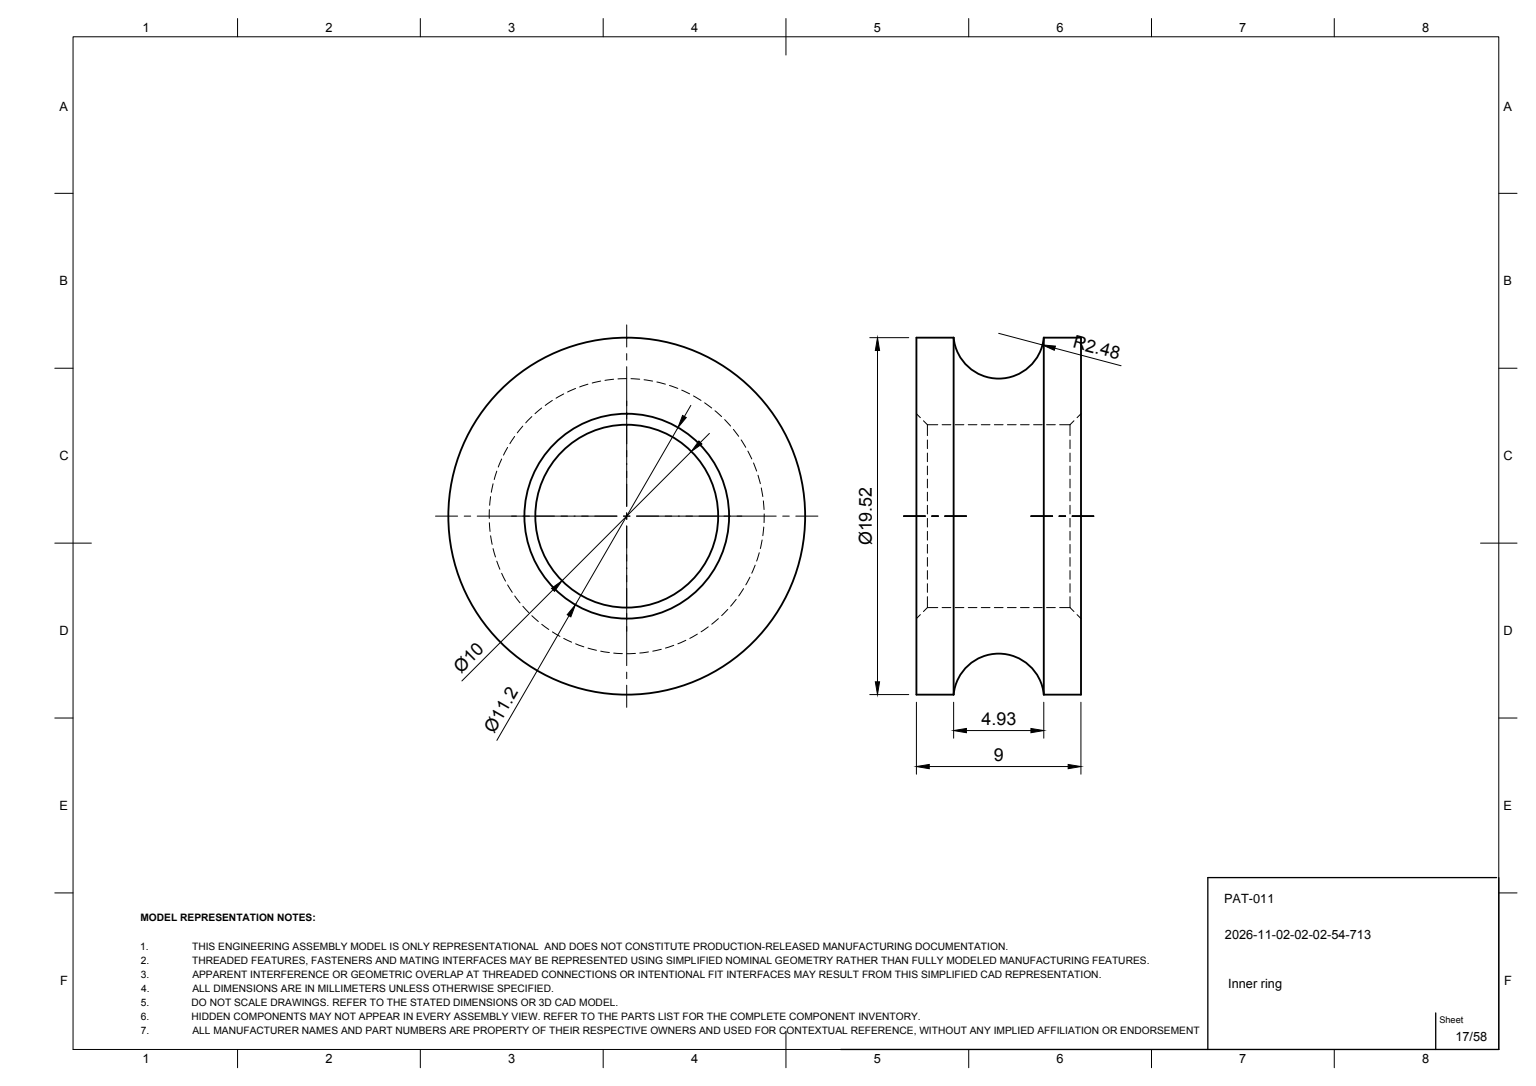
ISO-10303-21;
HEADER;
/* Generated by software containing ST-Developer
 * from STEP Tools, Inc. (www.steptools.com) 
 */

FILE_DESCRIPTION(
/* description */ ('Belt tension measurement rig'),
/* implementation_level */ '2;1');

FILE_NAME(
/* name */ 'Inner ring.step',
/* time_stamp */ '2026-10-28T03:24:44-07:00',
/* author */ (''),
/* organization */ (''),
/* preprocessor_version */ 'ST-DEVELOPER v20.2',
/* originating_system */ 'Autodesk Translation Framework v15.17.0.0',
/* authorisation */ '');

FILE_SCHEMA (('AUTOMOTIVE_DESIGN { 1 0 10303 214 3 1 1 }'));
ENDSEC;

DATA;
#10=MECHANICAL_DESIGN_GEOMETRIC_PRESENTATION_REPRESENTATION('',(#706),#23587);
#467=CONICAL_SURFACE('',#13234,0.53,0.785398163397448);
#468=CONICAL_SURFACE('',#13241,0.53,0.785398163397448);
#487=TOROIDAL_SURFACE('',#13223,1.,0.247676);
#596=SHAPE_REPRESENTATION_RELATIONSHIP('SRR','None',#23842,#651);
#651=ADVANCED_BREP_SHAPE_REPRESENTATION('',(#776),#23540);
#706=STYLED_ITEM('',(#24211),#776);
#776=MANIFOLD_SOLID_BREP('Body1',#12211);
#907=FACE_BOUND('',#2316,.T.);
#908=FACE_BOUND('',#2319,.T.);
#1138=PLANE('',#13236);
#1139=PLANE('',#13239);
#1529=FACE_OUTER_BOUND('',#2311,.T.);
#1530=FACE_OUTER_BOUND('',#2312,.T.);
#1531=FACE_OUTER_BOUND('',#2313,.T.);
#1532=FACE_OUTER_BOUND('',#2314,.T.);
#1533=FACE_OUTER_BOUND('',#2315,.T.);
#1534=FACE_OUTER_BOUND('',#2317,.T.);
#1535=FACE_OUTER_BOUND('',#2318,.T.);
#1536=FACE_OUTER_BOUND('',#2320,.T.);
#2311=EDGE_LOOP('',(#8684,#8685,#8686,#8687,#8688,#8689));
#2312=EDGE_LOOP('',(#8690,#8691,#8692,#8693,#8694));
#2313=EDGE_LOOP('',(#8695,#8696,#8697,#8698));
#2314=EDGE_LOOP('',(#8699,#8700,#8701,#8702));
#2315=EDGE_LOOP('',(#8703));
#2316=EDGE_LOOP('',(#8704));
#2317=EDGE_LOOP('',(#8705,#8706,#8707,#8708,#8709));
#2318=EDGE_LOOP('',(#8710));
#2319=EDGE_LOOP('',(#8711));
#2320=EDGE_LOOP('',(#8712,#8713,#8714,#8715));
#3185=LINE('',#19448,#3936);
#3186=LINE('',#19454,#3937);
#3187=LINE('',#19458,#3938);
#3188=LINE('',#19464,#3939);
#3189=LINE('',#19469,#3940);
#3936=VECTOR('',#15442,0.976185);
#3937=VECTOR('',#15449,0.5);
#3938=VECTOR('',#15454,0.53);
#3939=VECTOR('',#15463,0.976185);
#3940=VECTOR('',#15470,0.53);
#4622=CIRCLE('',#13224,0.976185);
#4623=CIRCLE('',#13225,0.976185);
#4624=CIRCLE('',#13226,0.247676);
#4625=CIRCLE('',#13227,0.976185);
#4626=CIRCLE('',#13228,0.976185);
#4627=CIRCLE('',#13230,0.976185);
#4628=CIRCLE('',#13232,0.5);
#4629=CIRCLE('',#13233,0.5);
#4630=CIRCLE('',#13235,0.56);
#4631=CIRCLE('',#13238,0.976185);
#4632=CIRCLE('',#13240,0.56);
#5484=VERTEX_POINT('',#19437);
#5485=VERTEX_POINT('',#19438);
#5486=VERTEX_POINT('',#19441);
#5487=VERTEX_POINT('',#19443);
#5488=VERTEX_POINT('',#19447);
#5489=VERTEX_POINT('',#19451);
#5490=VERTEX_POINT('',#19453);
#5491=VERTEX_POINT('',#19457);
#5492=VERTEX_POINT('',#19462);
#5493=VERTEX_POINT('',#19466);
#6701=EDGE_CURVE('',#5484,#5485,#4622,.T.);
#6702=EDGE_CURVE('',#5485,#5484,#4623,.T.);
#6703=EDGE_CURVE('',#5485,#5486,#4624,.T.);
#6704=EDGE_CURVE('',#5487,#5486,#4625,.T.);
#6705=EDGE_CURVE('',#5486,#5487,#4626,.T.);
#6706=EDGE_CURVE('',#5487,#5488,#3185,.T.);
#6707=EDGE_CURVE('',#5488,#5488,#4627,.T.);
#6708=EDGE_CURVE('',#5489,#5489,#4628,.T.);
#6709=EDGE_CURVE('',#5489,#5490,#3186,.T.);
#6710=EDGE_CURVE('',#5490,#5490,#4629,.T.);
#6711=EDGE_CURVE('',#5490,#5491,#3187,.T.);
#6712=EDGE_CURVE('',#5491,#5491,#4630,.T.);
#6713=EDGE_CURVE('',#5492,#5492,#4631,.T.);
#6714=EDGE_CURVE('',#5492,#5484,#3188,.T.);
#6715=EDGE_CURVE('',#5493,#5493,#4632,.T.);
#6716=EDGE_CURVE('',#5493,#5489,#3189,.T.);
#8684=ORIENTED_EDGE('',*,*,#6701,.F.);
#8685=ORIENTED_EDGE('',*,*,#6702,.F.);
#8686=ORIENTED_EDGE('',*,*,#6703,.T.);
#8687=ORIENTED_EDGE('',*,*,#6704,.F.);
#8688=ORIENTED_EDGE('',*,*,#6705,.F.);
#8689=ORIENTED_EDGE('',*,*,#6703,.F.);
#8690=ORIENTED_EDGE('',*,*,#6704,.T.);
#8691=ORIENTED_EDGE('',*,*,#6705,.T.);
#8692=ORIENTED_EDGE('',*,*,#6706,.T.);
#8693=ORIENTED_EDGE('',*,*,#6707,.T.);
#8694=ORIENTED_EDGE('',*,*,#6706,.F.);
#8695=ORIENTED_EDGE('',*,*,#6708,.T.);
#8696=ORIENTED_EDGE('',*,*,#6709,.T.);
#8697=ORIENTED_EDGE('',*,*,#6710,.F.);
#8698=ORIENTED_EDGE('',*,*,#6709,.F.);
#8699=ORIENTED_EDGE('',*,*,#6710,.T.);
#8700=ORIENTED_EDGE('',*,*,#6711,.T.);
#8701=ORIENTED_EDGE('',*,*,#6712,.F.);
#8702=ORIENTED_EDGE('',*,*,#6711,.F.);
#8703=ORIENTED_EDGE('',*,*,#6707,.F.);
#8704=ORIENTED_EDGE('',*,*,#6712,.T.);
#8705=ORIENTED_EDGE('',*,*,#6713,.F.);
#8706=ORIENTED_EDGE('',*,*,#6714,.T.);
#8707=ORIENTED_EDGE('',*,*,#6701,.T.);
#8708=ORIENTED_EDGE('',*,*,#6702,.T.);
#8709=ORIENTED_EDGE('',*,*,#6714,.F.);
#8710=ORIENTED_EDGE('',*,*,#6713,.T.);
#8711=ORIENTED_EDGE('',*,*,#6715,.F.);
#8712=ORIENTED_EDGE('',*,*,#6715,.T.);
#8713=ORIENTED_EDGE('',*,*,#6716,.T.);
#8714=ORIENTED_EDGE('',*,*,#6708,.F.);
#8715=ORIENTED_EDGE('',*,*,#6716,.F.);
#11234=CYLINDRICAL_SURFACE('',#13229,0.976185);
#11235=CYLINDRICAL_SURFACE('',#13231,0.5);
#11236=CYLINDRICAL_SURFACE('',#13237,0.976185);
#11670=ADVANCED_FACE('',(#1529),#487,.F.);
#11671=ADVANCED_FACE('',(#1530),#11234,.T.);
#11672=ADVANCED_FACE('',(#1531),#11235,.F.);
#11673=ADVANCED_FACE('',(#1532),#467,.F.);
#11674=ADVANCED_FACE('',(#1533,#907),#1138,.T.);
#11675=ADVANCED_FACE('',(#1534),#11236,.T.);
#11676=ADVANCED_FACE('',(#1535,#908),#1139,.T.);
#11677=ADVANCED_FACE('',(#1536),#468,.F.);
#12211=CLOSED_SHELL('',(#11670,#11671,#11672,#11673,#11674,#11675,#11676,
#11677));
#13222=AXIS2_PLACEMENT_3D('',#19435,#15426,#15427);
#13223=AXIS2_PLACEMENT_3D('',#19436,#15428,#15429);
#13224=AXIS2_PLACEMENT_3D('',#19439,#15430,#15431);
#13225=AXIS2_PLACEMENT_3D('',#19440,#15432,#15433);
#13226=AXIS2_PLACEMENT_3D('',#19442,#15434,#15435);
#13227=AXIS2_PLACEMENT_3D('',#19444,#15436,#15437);
#13228=AXIS2_PLACEMENT_3D('',#19445,#15438,#15439);
#13229=AXIS2_PLACEMENT_3D('',#19446,#15440,#15441);
#13230=AXIS2_PLACEMENT_3D('',#19449,#15443,#15444);
#13231=AXIS2_PLACEMENT_3D('',#19450,#15445,#15446);
#13232=AXIS2_PLACEMENT_3D('',#19452,#15447,#15448);
#13233=AXIS2_PLACEMENT_3D('',#19455,#15450,#15451);
#13234=AXIS2_PLACEMENT_3D('',#19456,#15452,#15453);
#13235=AXIS2_PLACEMENT_3D('',#19459,#15455,#15456);
#13236=AXIS2_PLACEMENT_3D('',#19460,#15457,#15458);
#13237=AXIS2_PLACEMENT_3D('',#19461,#15459,#15460);
#13238=AXIS2_PLACEMENT_3D('',#19463,#15461,#15462);
#13239=AXIS2_PLACEMENT_3D('',#19465,#15464,#15465);
#13240=AXIS2_PLACEMENT_3D('',#19467,#15466,#15467);
#13241=AXIS2_PLACEMENT_3D('',#19468,#15468,#15469);
#15426=DIRECTION('axis',(0.,0.,1.));
#15427=DIRECTION('refdir',(1.,0.,0.));
#15428=DIRECTION('center_axis',(0.,-1.,0.));
#15429=DIRECTION('ref_axis',(0.,0.,-1.));
#15430=DIRECTION('center_axis',(0.,-1.,0.));
#15431=DIRECTION('ref_axis',(1.,0.,0.));
#15432=DIRECTION('center_axis',(0.,-1.,0.));
#15433=DIRECTION('ref_axis',(1.,0.,0.));
#15434=DIRECTION('center_axis',(1.,0.,1.22464679914735E-16));
#15435=DIRECTION('ref_axis',(-1.22464679914735E-16,0.,1.));
#15436=DIRECTION('center_axis',(0.,1.,0.));
#15437=DIRECTION('ref_axis',(1.,0.,0.));
#15438=DIRECTION('center_axis',(0.,1.,0.));
#15439=DIRECTION('ref_axis',(1.,0.,0.));
#15440=DIRECTION('center_axis',(0.,-1.,0.));
#15441=DIRECTION('ref_axis',(1.,0.,0.));
#15442=DIRECTION('',(0.,1.,0.));
#15443=DIRECTION('center_axis',(0.,-1.,0.));
#15444=DIRECTION('ref_axis',(1.,0.,0.));
#15445=DIRECTION('center_axis',(0.,-1.,0.));
#15446=DIRECTION('ref_axis',(1.,0.,0.));
#15447=DIRECTION('center_axis',(0.,-1.,0.));
#15448=DIRECTION('ref_axis',(1.,0.,0.));
#15449=DIRECTION('',(0.,1.,0.));
#15450=DIRECTION('center_axis',(0.,-1.,0.));
#15451=DIRECTION('ref_axis',(1.,0.,0.));
#15452=DIRECTION('center_axis',(0.,1.,0.));
#15453=DIRECTION('ref_axis',(1.,0.,0.));
#15454=DIRECTION('',(-0.707106781186547,0.707106781186548,-8.65956056235493E-17));
#15455=DIRECTION('center_axis',(0.,-1.,0.));
#15456=DIRECTION('ref_axis',(1.,0.,0.));
#15457=DIRECTION('center_axis',(0.,1.,0.));
#15458=DIRECTION('ref_axis',(0.,0.,1.));
#15459=DIRECTION('center_axis',(0.,-1.,0.));
#15460=DIRECTION('ref_axis',(1.,0.,0.));
#15461=DIRECTION('center_axis',(0.,-1.,0.));
#15462=DIRECTION('ref_axis',(1.,0.,0.));
#15463=DIRECTION('',(0.,1.,0.));
#15464=DIRECTION('center_axis',(0.,-1.,0.));
#15465=DIRECTION('ref_axis',(0.,0.,-1.));
#15466=DIRECTION('center_axis',(0.,-1.,0.));
#15467=DIRECTION('ref_axis',(1.,0.,0.));
#15468=DIRECTION('center_axis',(0.,-1.,0.));
#15469=DIRECTION('ref_axis',(1.,0.,0.));
#15470=DIRECTION('',(0.707106781186547,0.707106781186548,8.65956056235493E-17));
#19435=CARTESIAN_POINT('',(0.,0.,0.));
#19436=CARTESIAN_POINT('Origin',(0.,0.,0.));
#19437=CARTESIAN_POINT('',(-0.976185,-0.246528389340863,-1.19548183562566E-16));
#19438=CARTESIAN_POINT('',(-1.19548183562566E-16,-0.246528389340863,0.976185));
#19439=CARTESIAN_POINT('Origin',(0.,-0.246528389340863,0.));
#19440=CARTESIAN_POINT('Origin',(0.,-0.246528389340863,0.));
#19441=CARTESIAN_POINT('',(-1.19548183562566E-16,0.246528389340863,0.976185));
#19442=CARTESIAN_POINT('Origin',(-1.22464679914735E-16,0.,1.));
#19443=CARTESIAN_POINT('',(-0.976185,0.246528389340863,1.19548183562566E-16));
#19444=CARTESIAN_POINT('Origin',(0.,0.246528389340863,0.));
#19445=CARTESIAN_POINT('Origin',(0.,0.246528389340863,0.));
#19446=CARTESIAN_POINT('Origin',(0.,0.,0.));
#19447=CARTESIAN_POINT('',(-0.976185,0.45,-1.19548183562566E-16));
#19448=CARTESIAN_POINT('',(-0.976185,0.,-1.19548183562566E-16));
#19449=CARTESIAN_POINT('Origin',(0.,0.45,0.));
#19450=CARTESIAN_POINT('Origin',(0.,0.,0.));
#19451=CARTESIAN_POINT('',(-0.5,-0.39,-6.12323399573677E-17));
#19452=CARTESIAN_POINT('Origin',(0.,-0.39,0.));
#19453=CARTESIAN_POINT('',(-0.5,0.39,-6.12323399573677E-17));
#19454=CARTESIAN_POINT('',(-0.5,0.,-6.12323399573677E-17));
#19455=CARTESIAN_POINT('Origin',(0.,0.39,0.));
#19456=CARTESIAN_POINT('Origin',(0.,0.42,0.));
#19457=CARTESIAN_POINT('',(-0.56,0.45,-6.85802207522518E-17));
#19458=CARTESIAN_POINT('',(-0.53,0.42,-6.49062803548097E-17));
#19459=CARTESIAN_POINT('Origin',(0.,0.45,0.));
#19460=CARTESIAN_POINT('Origin',(0.976185,0.45,0.));
#19461=CARTESIAN_POINT('Origin',(0.,0.,0.));
#19462=CARTESIAN_POINT('',(-0.976185,-0.45,-1.19548183562566E-16));
#19463=CARTESIAN_POINT('Origin',(0.,-0.45,0.));
#19464=CARTESIAN_POINT('',(-0.976185,0.,-1.19548183562566E-16));
#19465=CARTESIAN_POINT('Origin',(0.56,-0.45,0.));
#19466=CARTESIAN_POINT('',(-0.56,-0.45,-6.85802207522518E-17));
#19467=CARTESIAN_POINT('Origin',(0.,-0.45,0.));
#19468=CARTESIAN_POINT('Origin',(0.,-0.42,0.));
#19469=CARTESIAN_POINT('',(-0.53,-0.42,-6.49062803548097E-17));
#23475=UNCERTAINTY_MEASURE_WITH_UNIT(LENGTH_MEASURE(0.001),#23588,
'DISTANCE_ACCURACY_VALUE',
'Maximum model space distance between geometric entities at asserted c
onnectivities');
#23522=UNCERTAINTY_MEASURE_WITH_UNIT(LENGTH_MEASURE(0.001),#23588,
'DISTANCE_ACCURACY_VALUE',
'Maximum model space distance between geometric entities at asserted c
onnectivities');
#23540=(
GEOMETRIC_REPRESENTATION_CONTEXT(3)
GLOBAL_UNCERTAINTY_ASSIGNED_CONTEXT((#23475))
GLOBAL_UNIT_ASSIGNED_CONTEXT((#23588,#23590,#23591))
REPRESENTATION_CONTEXT('','3D')
);
#23587=(
GEOMETRIC_REPRESENTATION_CONTEXT(3)
GLOBAL_UNCERTAINTY_ASSIGNED_CONTEXT((#23522))
GLOBAL_UNIT_ASSIGNED_CONTEXT((#23588,#23590,#23591))
REPRESENTATION_CONTEXT('','3D')
);
#23588=(
LENGTH_UNIT()
NAMED_UNIT(*)
SI_UNIT(.CENTI.,.METRE.)
);
#23590=(
NAMED_UNIT(*)
PLANE_ANGLE_UNIT()
SI_UNIT($,.RADIAN.)
);
#23591=(
NAMED_UNIT(*)
SI_UNIT($,.STERADIAN.)
SOLID_ANGLE_UNIT()
);
#23609=SHAPE_DEFINITION_REPRESENTATION(#23673,#23842);
#23673=PRODUCT_DEFINITION_SHAPE('',$,#23907);
#23842=SHAPE_REPRESENTATION('',(#13222),#23540);
#23889=PRODUCT_DEFINITION_CONTEXT('part definition',#24083,'design');
#23907=PRODUCT_DEFINITION('Inner ring','Inner ring',#23971,#23889);
#23971=PRODUCT_DEFINITION_FORMATION('',$,#24102);
#24083=APPLICATION_CONTEXT(
'Core Data for Automotive Mechanical Design Process');
#24084=PRODUCT_CONTEXT('part definition',#24083,'mechanical');
#24102=PRODUCT('Inner ring','Inner ring','Inner ring',(#24084));
#24205=COLOUR_RGB('Grey',0.48,0.52,0.57);
#24206=FILL_AREA_STYLE_COLOUR('',#24205);
#24207=FILL_AREA_STYLE('',(#24206));
#24208=SURFACE_STYLE_FILL_AREA(#24207);
#24209=SURFACE_SIDE_STYLE('',(#24208));
#24210=SURFACE_STYLE_USAGE(.BOTH.,#24209);
#24211=PRESENTATION_STYLE_ASSIGNMENT((#24210));
ENDSEC;
END-ISO-10303-21;
